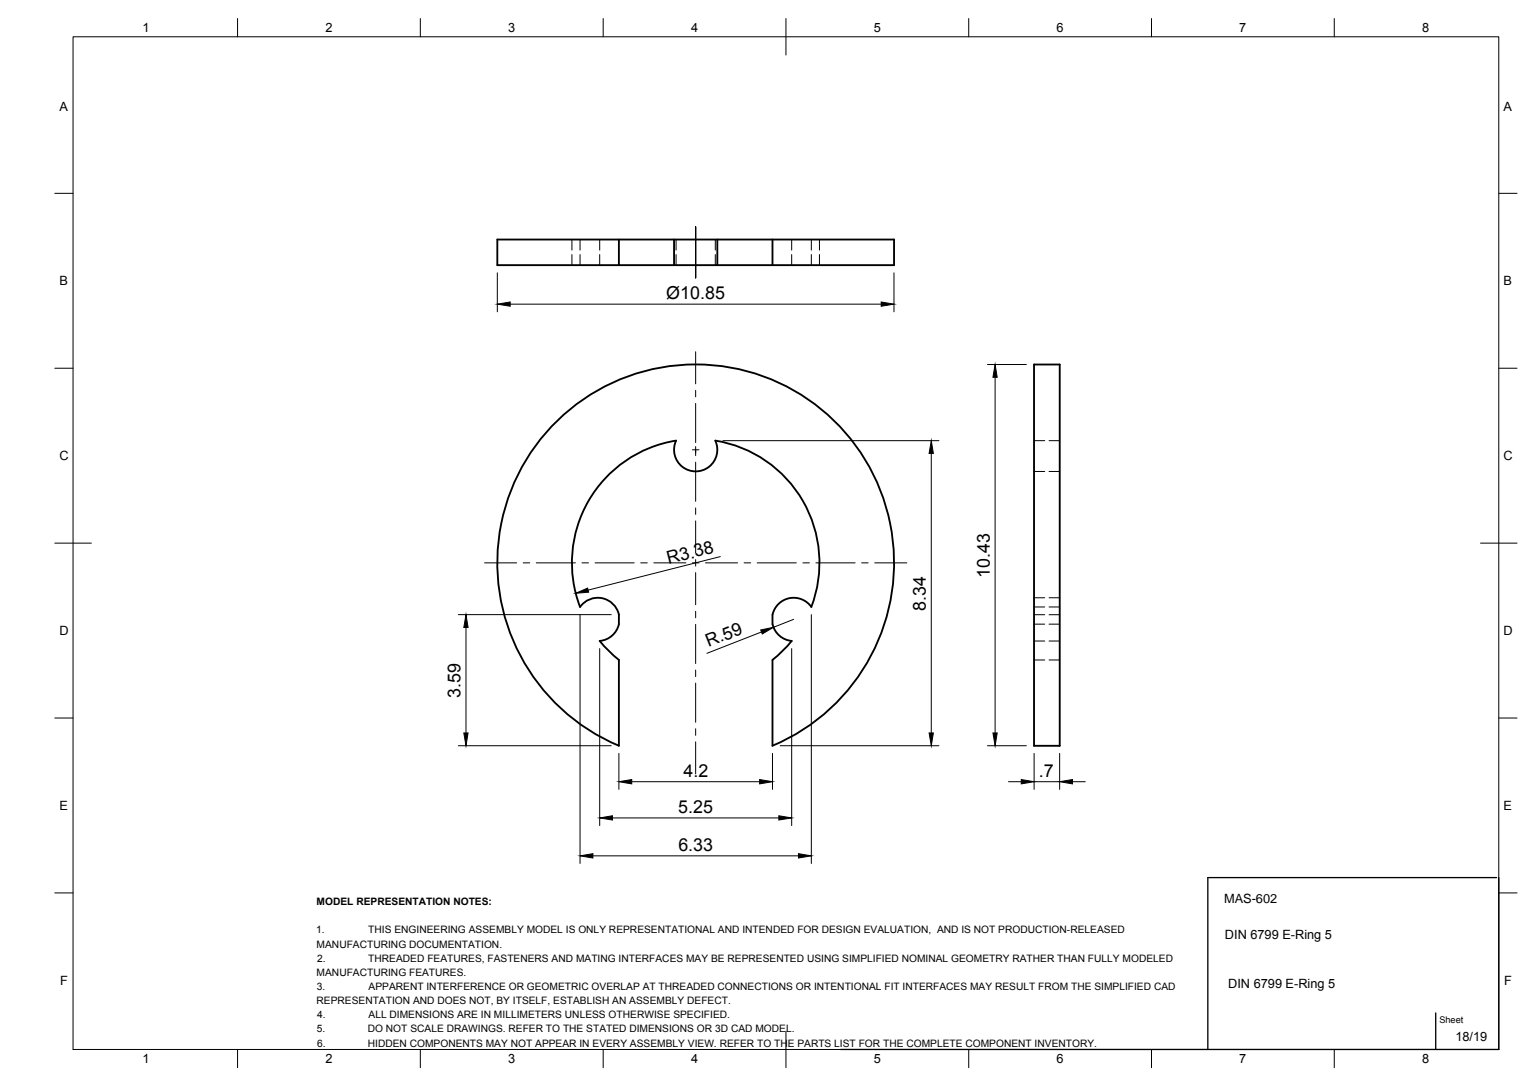
ISO-10303-21;
HEADER;
/* Generated by software containing ST-Developer
 * from STEP Tools, Inc. (www.steptools.com) 
 */

FILE_DESCRIPTION(
/* description */ (''),
/* implementation_level */ '2;1');

FILE_NAME(
/* name */ 'DIN 6799 E-Ring 5.step',
/* time_stamp */ '2026-10-15T14:42:47-07:00',
/* author */ (''),
/* organization */ (''),
/* preprocessor_version */ 'ST-DEVELOPER v20.2',
/* originating_system */ 'Autodesk Translation Framework v15.15.0.0',
/* authorisation */ '');

FILE_SCHEMA (('AUTOMOTIVE_DESIGN { 1 0 10303 214 3 1 1 }'));
ENDSEC;

DATA;
#10=MECHANICAL_DESIGN_GEOMETRIC_PRESENTATION_REPRESENTATION('',(#250),#85789);
#214=SHAPE_REPRESENTATION_RELATIONSHIP('SRR','None',#85879,#232);
#232=ADVANCED_BREP_SHAPE_REPRESENTATION('',(#268),#85787);
#250=STYLED_ITEM('',(#85978),#268);
#268=MANIFOLD_SOLID_BREP('Body1',#9897);
#1187=PLANE('',#10856);
#1188=PLANE('',#10857);
#1189=PLANE('',#10858);
#1190=PLANE('',#10859);
#1191=PLANE('',#10875);
#1192=PLANE('',#10891);
#1691=LINE('',#85550,#2227);
#1692=LINE('',#85552,#2228);
#1693=LINE('',#85554,#2229);
#1694=LINE('',#85555,#2230);
#1695=LINE('',#85559,#2231);
#1696=LINE('',#85561,#2232);
#1697=LINE('',#85563,#2233);
#1698=LINE('',#85564,#2234);
#1699=LINE('',#85568,#2235);
#1700=LINE('',#85570,#2236);
#1701=LINE('',#85572,#2237);
#1702=LINE('',#85573,#2238);
#1703=LINE('',#85577,#2239);
#1704=LINE('',#85579,#2240);
#1705=LINE('',#85581,#2241);
#1706=LINE('',#85582,#2242);
#1707=LINE('',#85587,#2243);
#1708=LINE('',#85593,#2244);
#1709=LINE('',#85599,#2245);
#1710=LINE('',#85605,#2246);
#1711=LINE('',#85623,#2247);
#1712=LINE('',#85627,#2248);
#2227=VECTOR('',#12969,1.);
#2228=VECTOR('',#12970,1.);
#2229=VECTOR('',#12971,1.);
#2230=VECTOR('',#12972,1.);
#2231=VECTOR('',#12975,1.);
#2232=VECTOR('',#12976,1.);
#2233=VECTOR('',#12977,1.);
#2234=VECTOR('',#12978,1.);
#2235=VECTOR('',#12981,1.);
#2236=VECTOR('',#12982,1.);
#2237=VECTOR('',#12983,1.);
#2238=VECTOR('',#12984,1.);
#2239=VECTOR('',#12987,1.);
#2240=VECTOR('',#12988,1.);
#2241=VECTOR('',#12989,1.);
#2242=VECTOR('',#12990,1.);
#2243=VECTOR('',#12995,1.);
#2244=VECTOR('',#13002,1.);
#2245=VECTOR('',#13009,1.);
#2246=VECTOR('',#13016,1.);
#2247=VECTOR('',#13045,1.);
#2248=VECTOR('',#13050,1.);
#2382=CYLINDRICAL_SURFACE('',#10860,0.059240625);
#2383=CYLINDRICAL_SURFACE('',#10863,0.059240625);
#2384=CYLINDRICAL_SURFACE('',#10866,0.059240625);
#2385=CYLINDRICAL_SURFACE('',#10869,0.059240625);
#2386=CYLINDRICAL_SURFACE('',#10872,0.33848125);
#2387=CYLINDRICAL_SURFACE('',#10881,0.33848125);
#2388=CYLINDRICAL_SURFACE('',#10883,0.33848125);
#2389=CYLINDRICAL_SURFACE('',#10885,0.059240625);
#2390=CYLINDRICAL_SURFACE('',#10887,0.33848125);
#2391=CYLINDRICAL_SURFACE('',#10889,0.5425);
#2871=FACE_OUTER_BOUND('',#3461,.T.);
#2872=FACE_OUTER_BOUND('',#3462,.T.);
#2873=FACE_OUTER_BOUND('',#3463,.T.);
#2874=FACE_OUTER_BOUND('',#3464,.T.);
#2875=FACE_OUTER_BOUND('',#3465,.T.);
#2876=FACE_OUTER_BOUND('',#3466,.T.);
#2877=FACE_OUTER_BOUND('',#3467,.T.);
#2878=FACE_OUTER_BOUND('',#3468,.T.);
#2879=FACE_OUTER_BOUND('',#3469,.T.);
#2880=FACE_OUTER_BOUND('',#3470,.T.);
#2881=FACE_OUTER_BOUND('',#3471,.T.);
#2882=FACE_OUTER_BOUND('',#3472,.T.);
#2883=FACE_OUTER_BOUND('',#3473,.T.);
#2884=FACE_OUTER_BOUND('',#3474,.T.);
#2885=FACE_OUTER_BOUND('',#3475,.T.);
#2886=FACE_OUTER_BOUND('',#3476,.T.);
#3461=EDGE_LOOP('',(#9207,#9208,#9209,#9210));
#3462=EDGE_LOOP('',(#9211,#9212,#9213,#9214));
#3463=EDGE_LOOP('',(#9215,#9216,#9217,#9218));
#3464=EDGE_LOOP('',(#9219,#9220,#9221,#9222));
#3465=EDGE_LOOP('',(#9223,#9224,#9225,#9226));
#3466=EDGE_LOOP('',(#9227,#9228,#9229,#9230));
#3467=EDGE_LOOP('',(#9231,#9232,#9233,#9234));
#3468=EDGE_LOOP('',(#9235,#9236,#9237,#9238));
#3469=EDGE_LOOP('',(#9239,#9240,#9241,#9242));
#3470=EDGE_LOOP('',(#9243,#9244,#9245,#9246,#9247,#9248,#9249,#9250,#9251,
#9252,#9253,#9254,#9255,#9256));
#3471=EDGE_LOOP('',(#9257,#9258,#9259,#9260));
#3472=EDGE_LOOP('',(#9261,#9262,#9263,#9264));
#3473=EDGE_LOOP('',(#9265,#9266,#9267,#9268));
#3474=EDGE_LOOP('',(#9269,#9270,#9271,#9272));
#3475=EDGE_LOOP('',(#9273,#9274,#9275,#9276));
#3476=EDGE_LOOP('',(#9277,#9278,#9279,#9280,#9281,#9282,#9283,#9284,#9285,
#9286,#9287,#9288,#9289,#9290));
#3855=CIRCLE('',#10861,0.059240625);
#3856=CIRCLE('',#10862,0.059240625);
#3857=CIRCLE('',#10864,0.059240625);
#3858=CIRCLE('',#10865,0.059240625);
#3859=CIRCLE('',#10867,0.059240625);
#3860=CIRCLE('',#10868,0.059240625);
#3861=CIRCLE('',#10870,0.059240625);
#3862=CIRCLE('',#10871,0.059240625);
#3863=CIRCLE('',#10873,0.33848125);
#3864=CIRCLE('',#10874,0.33848125);
#3865=CIRCLE('',#10876,0.33848125);
#3866=CIRCLE('',#10877,0.059240625);
#3867=CIRCLE('',#10878,0.33848125);
#3868=CIRCLE('',#10879,0.5425);
#3869=CIRCLE('',#10880,0.33848125);
#3870=CIRCLE('',#10882,0.33848125);
#3871=CIRCLE('',#10884,0.33848125);
#3872=CIRCLE('',#10886,0.059240625);
#3873=CIRCLE('',#10888,0.33848125);
#3874=CIRCLE('',#10890,0.5425);
#4879=VERTEX_POINT('',#85548);
#4880=VERTEX_POINT('',#85549);
#4881=VERTEX_POINT('',#85551);
#4882=VERTEX_POINT('',#85553);
#4883=VERTEX_POINT('',#85557);
#4884=VERTEX_POINT('',#85558);
#4885=VERTEX_POINT('',#85560);
#4886=VERTEX_POINT('',#85562);
#4887=VERTEX_POINT('',#85566);
#4888=VERTEX_POINT('',#85567);
#4889=VERTEX_POINT('',#85569);
#4890=VERTEX_POINT('',#85571);
#4891=VERTEX_POINT('',#85575);
#4892=VERTEX_POINT('',#85576);
#4893=VERTEX_POINT('',#85578);
#4894=VERTEX_POINT('',#85580);
#4895=VERTEX_POINT('',#85584);
#4896=VERTEX_POINT('',#85586);
#4897=VERTEX_POINT('',#85590);
#4898=VERTEX_POINT('',#85592);
#4899=VERTEX_POINT('',#85596);
#4900=VERTEX_POINT('',#85598);
#4901=VERTEX_POINT('',#85602);
#4902=VERTEX_POINT('',#85604);
#4903=VERTEX_POINT('',#85611);
#4904=VERTEX_POINT('',#85613);
#4905=VERTEX_POINT('',#85621);
#4906=VERTEX_POINT('',#85625);
#6331=EDGE_CURVE('',#4879,#4880,#1691,.T.);
#6332=EDGE_CURVE('',#4881,#4879,#1692,.T.);
#6333=EDGE_CURVE('',#4882,#4881,#1693,.T.);
#6334=EDGE_CURVE('',#4880,#4882,#1694,.T.);
#6335=EDGE_CURVE('',#4883,#4884,#1695,.T.);
#6336=EDGE_CURVE('',#4885,#4883,#1696,.T.);
#6337=EDGE_CURVE('',#4886,#4885,#1697,.T.);
#6338=EDGE_CURVE('',#4884,#4886,#1698,.T.);
#6339=EDGE_CURVE('',#4887,#4888,#1699,.T.);
#6340=EDGE_CURVE('',#4889,#4887,#1700,.T.);
#6341=EDGE_CURVE('',#4890,#4889,#1701,.T.);
#6342=EDGE_CURVE('',#4888,#4890,#1702,.T.);
#6343=EDGE_CURVE('',#4891,#4892,#1703,.T.);
#6344=EDGE_CURVE('',#4893,#4891,#1704,.T.);
#6345=EDGE_CURVE('',#4894,#4893,#1705,.T.);
#6346=EDGE_CURVE('',#4892,#4894,#1706,.T.);
#6347=EDGE_CURVE('',#4895,#4885,#3855,.T.);
#6348=EDGE_CURVE('',#4896,#4895,#1707,.T.);
#6349=EDGE_CURVE('',#4896,#4886,#3856,.T.);
#6350=EDGE_CURVE('',#4884,#4897,#3857,.T.);
#6351=EDGE_CURVE('',#4897,#4898,#1708,.T.);
#6352=EDGE_CURVE('',#4883,#4898,#3858,.T.);
#6353=EDGE_CURVE('',#4899,#4893,#3859,.T.);
#6354=EDGE_CURVE('',#4900,#4899,#1709,.T.);
#6355=EDGE_CURVE('',#4900,#4894,#3860,.T.);
#6356=EDGE_CURVE('',#4892,#4901,#3861,.T.);
#6357=EDGE_CURVE('',#4901,#4902,#1710,.T.);
#6358=EDGE_CURVE('',#4891,#4902,#3862,.T.);
#6359=EDGE_CURVE('',#4888,#4900,#3863,.T.);
#6360=EDGE_CURVE('',#4887,#4899,#3864,.T.);
#6361=EDGE_CURVE('',#4903,#4896,#3865,.T.);
#6362=EDGE_CURVE('',#4904,#4903,#3866,.T.);
#6363=EDGE_CURVE('',#4901,#4904,#3867,.T.);
#6364=EDGE_CURVE('',#4881,#4890,#3868,.T.);
#6365=EDGE_CURVE('',#4897,#4879,#3869,.T.);
#6366=EDGE_CURVE('',#4898,#4880,#3870,.T.);
#6367=EDGE_CURVE('',#4905,#4895,#3871,.T.);
#6368=EDGE_CURVE('',#4903,#4905,#1711,.T.);
#6369=EDGE_CURVE('',#4906,#4905,#3872,.T.);
#6370=EDGE_CURVE('',#4904,#4906,#1712,.T.);
#6371=EDGE_CURVE('',#4902,#4906,#3873,.T.);
#6372=EDGE_CURVE('',#4882,#4889,#3874,.T.);
#9207=ORIENTED_EDGE('',*,*,#6331,.F.);
#9208=ORIENTED_EDGE('',*,*,#6332,.F.);
#9209=ORIENTED_EDGE('',*,*,#6333,.F.);
#9210=ORIENTED_EDGE('',*,*,#6334,.F.);
#9211=ORIENTED_EDGE('',*,*,#6335,.F.);
#9212=ORIENTED_EDGE('',*,*,#6336,.F.);
#9213=ORIENTED_EDGE('',*,*,#6337,.F.);
#9214=ORIENTED_EDGE('',*,*,#6338,.F.);
#9215=ORIENTED_EDGE('',*,*,#6339,.F.);
#9216=ORIENTED_EDGE('',*,*,#6340,.F.);
#9217=ORIENTED_EDGE('',*,*,#6341,.F.);
#9218=ORIENTED_EDGE('',*,*,#6342,.F.);
#9219=ORIENTED_EDGE('',*,*,#6343,.F.);
#9220=ORIENTED_EDGE('',*,*,#6344,.F.);
#9221=ORIENTED_EDGE('',*,*,#6345,.F.);
#9222=ORIENTED_EDGE('',*,*,#6346,.F.);
#9223=ORIENTED_EDGE('',*,*,#6337,.T.);
#9224=ORIENTED_EDGE('',*,*,#6347,.F.);
#9225=ORIENTED_EDGE('',*,*,#6348,.F.);
#9226=ORIENTED_EDGE('',*,*,#6349,.T.);
#9227=ORIENTED_EDGE('',*,*,#6335,.T.);
#9228=ORIENTED_EDGE('',*,*,#6350,.T.);
#9229=ORIENTED_EDGE('',*,*,#6351,.T.);
#9230=ORIENTED_EDGE('',*,*,#6352,.F.);
#9231=ORIENTED_EDGE('',*,*,#6345,.T.);
#9232=ORIENTED_EDGE('',*,*,#6353,.F.);
#9233=ORIENTED_EDGE('',*,*,#6354,.F.);
#9234=ORIENTED_EDGE('',*,*,#6355,.T.);
#9235=ORIENTED_EDGE('',*,*,#6343,.T.);
#9236=ORIENTED_EDGE('',*,*,#6356,.T.);
#9237=ORIENTED_EDGE('',*,*,#6357,.T.);
#9238=ORIENTED_EDGE('',*,*,#6358,.F.);
#9239=ORIENTED_EDGE('',*,*,#6339,.T.);
#9240=ORIENTED_EDGE('',*,*,#6359,.T.);
#9241=ORIENTED_EDGE('',*,*,#6354,.T.);
#9242=ORIENTED_EDGE('',*,*,#6360,.F.);
#9243=ORIENTED_EDGE('',*,*,#6338,.T.);
#9244=ORIENTED_EDGE('',*,*,#6349,.F.);
#9245=ORIENTED_EDGE('',*,*,#6361,.F.);
#9246=ORIENTED_EDGE('',*,*,#6362,.F.);
#9247=ORIENTED_EDGE('',*,*,#6363,.F.);
#9248=ORIENTED_EDGE('',*,*,#6356,.F.);
#9249=ORIENTED_EDGE('',*,*,#6346,.T.);
#9250=ORIENTED_EDGE('',*,*,#6355,.F.);
#9251=ORIENTED_EDGE('',*,*,#6359,.F.);
#9252=ORIENTED_EDGE('',*,*,#6342,.T.);
#9253=ORIENTED_EDGE('',*,*,#6364,.F.);
#9254=ORIENTED_EDGE('',*,*,#6332,.T.);
#9255=ORIENTED_EDGE('',*,*,#6365,.F.);
#9256=ORIENTED_EDGE('',*,*,#6350,.F.);
#9257=ORIENTED_EDGE('',*,*,#6331,.T.);
#9258=ORIENTED_EDGE('',*,*,#6366,.F.);
#9259=ORIENTED_EDGE('',*,*,#6351,.F.);
#9260=ORIENTED_EDGE('',*,*,#6365,.T.);
#9261=ORIENTED_EDGE('',*,*,#6361,.T.);
#9262=ORIENTED_EDGE('',*,*,#6348,.T.);
#9263=ORIENTED_EDGE('',*,*,#6367,.F.);
#9264=ORIENTED_EDGE('',*,*,#6368,.F.);
#9265=ORIENTED_EDGE('',*,*,#6362,.T.);
#9266=ORIENTED_EDGE('',*,*,#6368,.T.);
#9267=ORIENTED_EDGE('',*,*,#6369,.F.);
#9268=ORIENTED_EDGE('',*,*,#6370,.F.);
#9269=ORIENTED_EDGE('',*,*,#6363,.T.);
#9270=ORIENTED_EDGE('',*,*,#6370,.T.);
#9271=ORIENTED_EDGE('',*,*,#6371,.F.);
#9272=ORIENTED_EDGE('',*,*,#6357,.F.);
#9273=ORIENTED_EDGE('',*,*,#6333,.T.);
#9274=ORIENTED_EDGE('',*,*,#6364,.T.);
#9275=ORIENTED_EDGE('',*,*,#6341,.T.);
#9276=ORIENTED_EDGE('',*,*,#6372,.F.);
#9277=ORIENTED_EDGE('',*,*,#6336,.T.);
#9278=ORIENTED_EDGE('',*,*,#6352,.T.);
#9279=ORIENTED_EDGE('',*,*,#6366,.T.);
#9280=ORIENTED_EDGE('',*,*,#6334,.T.);
#9281=ORIENTED_EDGE('',*,*,#6372,.T.);
#9282=ORIENTED_EDGE('',*,*,#6340,.T.);
#9283=ORIENTED_EDGE('',*,*,#6360,.T.);
#9284=ORIENTED_EDGE('',*,*,#6353,.T.);
#9285=ORIENTED_EDGE('',*,*,#6344,.T.);
#9286=ORIENTED_EDGE('',*,*,#6358,.T.);
#9287=ORIENTED_EDGE('',*,*,#6371,.T.);
#9288=ORIENTED_EDGE('',*,*,#6369,.T.);
#9289=ORIENTED_EDGE('',*,*,#6367,.T.);
#9290=ORIENTED_EDGE('',*,*,#6347,.T.);
#9849=ADVANCED_FACE('',(#2871),#1187,.F.);
#9850=ADVANCED_FACE('',(#2872),#1188,.F.);
#9851=ADVANCED_FACE('',(#2873),#1189,.F.);
#9852=ADVANCED_FACE('',(#2874),#1190,.F.);
#9853=ADVANCED_FACE('',(#2875),#2382,.T.);
#9854=ADVANCED_FACE('',(#2876),#2383,.T.);
#9855=ADVANCED_FACE('',(#2877),#2384,.T.);
#9856=ADVANCED_FACE('',(#2878),#2385,.T.);
#9857=ADVANCED_FACE('',(#2879),#2386,.F.);
#9858=ADVANCED_FACE('',(#2880),#1191,.F.);
#9859=ADVANCED_FACE('',(#2881),#2387,.F.);
#9860=ADVANCED_FACE('',(#2882),#2388,.F.);
#9861=ADVANCED_FACE('',(#2883),#2389,.T.);
#9862=ADVANCED_FACE('',(#2884),#2390,.F.);
#9863=ADVANCED_FACE('',(#2885),#2391,.T.);
#9864=ADVANCED_FACE('',(#2886),#1192,.T.);
#9897=CLOSED_SHELL('',(#9849,#9850,#9851,#9852,#9853,#9854,#9855,#9856,
#9857,#9858,#9859,#9860,#9861,#9862,#9863,#9864));
#10855=AXIS2_PLACEMENT_3D('',#85546,#12965,#12966);
#10856=AXIS2_PLACEMENT_3D('',#85547,#12967,#12968);
#10857=AXIS2_PLACEMENT_3D('',#85556,#12973,#12974);
#10858=AXIS2_PLACEMENT_3D('',#85565,#12979,#12980);
#10859=AXIS2_PLACEMENT_3D('',#85574,#12985,#12986);
#10860=AXIS2_PLACEMENT_3D('',#85583,#12991,#12992);
#10861=AXIS2_PLACEMENT_3D('',#85585,#12993,#12994);
#10862=AXIS2_PLACEMENT_3D('',#85588,#12996,#12997);
#10863=AXIS2_PLACEMENT_3D('',#85589,#12998,#12999);
#10864=AXIS2_PLACEMENT_3D('',#85591,#13000,#13001);
#10865=AXIS2_PLACEMENT_3D('',#85594,#13003,#13004);
#10866=AXIS2_PLACEMENT_3D('',#85595,#13005,#13006);
#10867=AXIS2_PLACEMENT_3D('',#85597,#13007,#13008);
#10868=AXIS2_PLACEMENT_3D('',#85600,#13010,#13011);
#10869=AXIS2_PLACEMENT_3D('',#85601,#13012,#13013);
#10870=AXIS2_PLACEMENT_3D('',#85603,#13014,#13015);
#10871=AXIS2_PLACEMENT_3D('',#85606,#13017,#13018);
#10872=AXIS2_PLACEMENT_3D('',#85607,#13019,#13020);
#10873=AXIS2_PLACEMENT_3D('',#85608,#13021,#13022);
#10874=AXIS2_PLACEMENT_3D('',#85609,#13023,#13024);
#10875=AXIS2_PLACEMENT_3D('',#85610,#13025,#13026);
#10876=AXIS2_PLACEMENT_3D('',#85612,#13027,#13028);
#10877=AXIS2_PLACEMENT_3D('',#85614,#13029,#13030);
#10878=AXIS2_PLACEMENT_3D('',#85615,#13031,#13032);
#10879=AXIS2_PLACEMENT_3D('',#85616,#13033,#13034);
#10880=AXIS2_PLACEMENT_3D('',#85617,#13035,#13036);
#10881=AXIS2_PLACEMENT_3D('',#85618,#13037,#13038);
#10882=AXIS2_PLACEMENT_3D('',#85619,#13039,#13040);
#10883=AXIS2_PLACEMENT_3D('',#85620,#13041,#13042);
#10884=AXIS2_PLACEMENT_3D('',#85622,#13043,#13044);
#10885=AXIS2_PLACEMENT_3D('',#85624,#13046,#13047);
#10886=AXIS2_PLACEMENT_3D('',#85626,#13048,#13049);
#10887=AXIS2_PLACEMENT_3D('',#85628,#13051,#13052);
#10888=AXIS2_PLACEMENT_3D('',#85629,#13053,#13054);
#10889=AXIS2_PLACEMENT_3D('',#85630,#13055,#13056);
#10890=AXIS2_PLACEMENT_3D('',#85631,#13057,#13058);
#10891=AXIS2_PLACEMENT_3D('',#85632,#13059,#13060);
#12965=DIRECTION('axis',(0.,0.,1.));
#12966=DIRECTION('refdir',(1.,0.,0.));
#12967=DIRECTION('center_axis',(0.,1.,0.));
#12968=DIRECTION('ref_axis',(0.,0.,1.));
#12969=DIRECTION('',(1.,0.,0.));
#12970=DIRECTION('',(0.,0.,1.));
#12971=DIRECTION('',(-1.,0.,0.));
#12972=DIRECTION('',(0.,0.,-1.));
#12973=DIRECTION('center_axis',(0.,1.,0.));
#12974=DIRECTION('ref_axis',(0.,0.,1.));
#12975=DIRECTION('',(-1.,0.,0.));
#12976=DIRECTION('',(0.,0.,-1.));
#12977=DIRECTION('',(1.,0.,0.));
#12978=DIRECTION('',(0.,0.,1.));
#12979=DIRECTION('center_axis',(0.,-1.,0.));
#12980=DIRECTION('ref_axis',(0.,0.,-1.));
#12981=DIRECTION('',(-1.,0.,0.));
#12982=DIRECTION('',(0.,0.,1.));
#12983=DIRECTION('',(1.,0.,0.));
#12984=DIRECTION('',(0.,0.,-1.));
#12985=DIRECTION('center_axis',(0.,-1.,0.));
#12986=DIRECTION('ref_axis',(0.,0.,-1.));
#12987=DIRECTION('',(-1.,0.,0.));
#12988=DIRECTION('',(0.,0.,1.));
#12989=DIRECTION('',(1.,0.,0.));
#12990=DIRECTION('',(0.,0.,-1.));
#12991=DIRECTION('center_axis',(1.,0.,0.));
#12992=DIRECTION('ref_axis',(0.,-0.194892865217565,0.980824536340363));
#12993=DIRECTION('center_axis',(1.,0.,0.));
#12994=DIRECTION('ref_axis',(0.,0.,-1.));
#12995=DIRECTION('',(1.,0.,0.));
#12996=DIRECTION('center_axis',(1.,0.,0.));
#12997=DIRECTION('ref_axis',(0.,0.,-1.));
#12998=DIRECTION('center_axis',(1.,0.,0.));
#12999=DIRECTION('ref_axis',(0.,0.,-1.));
#13000=DIRECTION('center_axis',(1.,0.,0.));
#13001=DIRECTION('ref_axis',(0.,0.,-1.));
#13002=DIRECTION('',(1.,0.,0.));
#13003=DIRECTION('center_axis',(1.,0.,0.));
#13004=DIRECTION('ref_axis',(0.,0.,-1.));
#13005=DIRECTION('center_axis',(1.,0.,0.));
#13006=DIRECTION('ref_axis',(0.,0.,-1.));
#13007=DIRECTION('center_axis',(1.,0.,0.));
#13008=DIRECTION('ref_axis',(0.,0.,-1.));
#13009=DIRECTION('',(1.,0.,0.));
#13010=DIRECTION('center_axis',(1.,0.,0.));
#13011=DIRECTION('ref_axis',(0.,0.,-1.));
#13012=DIRECTION('center_axis',(1.,0.,0.));
#13013=DIRECTION('ref_axis',(0.,0.194892865217571,0.980824536340362));
#13014=DIRECTION('center_axis',(1.,0.,0.));
#13015=DIRECTION('ref_axis',(0.,0.,-1.));
#13016=DIRECTION('',(1.,0.,0.));
#13017=DIRECTION('center_axis',(1.,0.,0.));
#13018=DIRECTION('ref_axis',(0.,0.,-1.));
#13019=DIRECTION('center_axis',(1.,0.,0.));
#13020=DIRECTION('ref_axis',(0.,0.,-1.));
#13021=DIRECTION('center_axis',(-1.,0.,0.));
#13022=DIRECTION('ref_axis',(0.,0.,-1.));
#13023=DIRECTION('center_axis',(-1.,0.,0.));
#13024=DIRECTION('ref_axis',(0.,0.,-1.));
#13025=DIRECTION('center_axis',(1.,0.,0.));
#13026=DIRECTION('ref_axis',(0.,0.,-1.));
#13027=DIRECTION('center_axis',(-1.,0.,0.));
#13028=DIRECTION('ref_axis',(0.,0.,-1.));
#13029=DIRECTION('center_axis',(1.,0.,0.));
#13030=DIRECTION('ref_axis',(0.,0.,-1.));
#13031=DIRECTION('center_axis',(-1.,0.,0.));
#13032=DIRECTION('ref_axis',(0.,0.,-1.));
#13033=DIRECTION('center_axis',(1.,0.,0.));
#13034=DIRECTION('ref_axis',(0.,0.,-1.));
#13035=DIRECTION('center_axis',(-1.,0.,0.));
#13036=DIRECTION('ref_axis',(0.,0.,-1.));
#13037=DIRECTION('center_axis',(1.,0.,0.));
#13038=DIRECTION('ref_axis',(0.,0.,-1.));
#13039=DIRECTION('center_axis',(-1.,0.,0.));
#13040=DIRECTION('ref_axis',(0.,0.,-1.));
#13041=DIRECTION('center_axis',(1.,0.,0.));
#13042=DIRECTION('ref_axis',(0.,0.,-1.));
#13043=DIRECTION('center_axis',(-1.,0.,0.));
#13044=DIRECTION('ref_axis',(0.,0.,-1.));
#13045=DIRECTION('',(1.,0.,0.));
#13046=DIRECTION('center_axis',(1.,0.,0.));
#13047=DIRECTION('ref_axis',(0.,0.,-1.));
#13048=DIRECTION('center_axis',(1.,0.,0.));
#13049=DIRECTION('ref_axis',(0.,0.,-1.));
#13050=DIRECTION('',(1.,0.,0.));
#13051=DIRECTION('center_axis',(1.,0.,0.));
#13052=DIRECTION('ref_axis',(0.,0.,-1.));
#13053=DIRECTION('center_axis',(-1.,0.,0.));
#13054=DIRECTION('ref_axis',(0.,0.,-1.));
#13055=DIRECTION('center_axis',(1.,0.,0.));
#13056=DIRECTION('ref_axis',(0.,1.22464679914735E-16,1.));
#13057=DIRECTION('center_axis',(1.,0.,0.));
#13058=DIRECTION('ref_axis',(0.,0.,-1.));
#13059=DIRECTION('center_axis',(1.,0.,0.));
#13060=DIRECTION('ref_axis',(0.,0.,-1.));
#85546=CARTESIAN_POINT('',(0.,0.,0.));
#85547=CARTESIAN_POINT('Origin',(0.,0.21,-1.085));
#85548=CARTESIAN_POINT('',(0.,0.21,-0.265461026520961));
#85549=CARTESIAN_POINT('',(0.07,0.21,-0.265461026520961));
#85550=CARTESIAN_POINT('',(0.,0.21,-0.265461026520961));
#85551=CARTESIAN_POINT('',(0.,0.21,-0.500206207478476));
#85552=CARTESIAN_POINT('',(0.,0.21,-0.5425));
#85553=CARTESIAN_POINT('',(0.07,0.21,-0.500206207478476));
#85554=CARTESIAN_POINT('',(0.,0.21,-0.500206207478476));
#85555=CARTESIAN_POINT('',(0.07,0.21,-0.5425));
#85556=CARTESIAN_POINT('Origin',(0.,0.21,-1.085));
#85557=CARTESIAN_POINT('',(0.07,0.21,-0.167559714847562));
#85558=CARTESIAN_POINT('',(0.,0.21,-0.167559714847562));
#85559=CARTESIAN_POINT('',(0.,0.21,-0.167559714847562));
#85560=CARTESIAN_POINT('',(0.07,0.21,-0.141680910152439));
#85561=CARTESIAN_POINT('',(0.07,0.21,-0.5425));
#85562=CARTESIAN_POINT('',(0.,0.21,-0.141680910152439));
#85563=CARTESIAN_POINT('',(0.,0.21,-0.141680910152439));
#85564=CARTESIAN_POINT('',(0.,0.21,-0.5425));
#85565=CARTESIAN_POINT('Origin',(0.,-0.21,-0.075));
#85566=CARTESIAN_POINT('',(0.07,-0.21,-0.265461026520961));
#85567=CARTESIAN_POINT('',(0.,-0.21,-0.265461026520961));
#85568=CARTESIAN_POINT('',(0.,-0.21,-0.265461026520961));
#85569=CARTESIAN_POINT('',(0.07,-0.21,-0.500206207478476));
#85570=CARTESIAN_POINT('',(0.07,-0.21,-0.0375));
#85571=CARTESIAN_POINT('',(0.,-0.21,-0.500206207478476));
#85572=CARTESIAN_POINT('',(0.,-0.21,-0.500206207478476));
#85573=CARTESIAN_POINT('',(0.,-0.21,-0.0375));
#85574=CARTESIAN_POINT('Origin',(0.,-0.21,-0.075));
#85575=CARTESIAN_POINT('',(0.07,-0.21,-0.141680910152439));
#85576=CARTESIAN_POINT('',(0.,-0.21,-0.141680910152439));
#85577=CARTESIAN_POINT('',(0.,-0.21,-0.141680910152439));
#85578=CARTESIAN_POINT('',(0.07,-0.21,-0.167559714847561));
#85579=CARTESIAN_POINT('',(0.07,-0.21,-0.0375));
#85580=CARTESIAN_POINT('',(0.,-0.21,-0.167559714847561));
#85581=CARTESIAN_POINT('',(0.,-0.21,-0.167559714847561));
#85582=CARTESIAN_POINT('',(0.,-0.21,-0.0375));
#85583=CARTESIAN_POINT('Origin',(0.,0.267810237132177,-0.1546203125));
#85584=CARTESIAN_POINT('',(0.07,0.31628195418898,-0.120562357541491));
#85585=CARTESIAN_POINT('Origin',(0.07,0.267810237132177,-0.1546203125));
#85586=CARTESIAN_POINT('',(0.,0.31628195418898,-0.120562357541491));
#85587=CARTESIAN_POINT('',(0.,0.31628195418898,-0.120562357541491));
#85588=CARTESIAN_POINT('Origin',(0.,0.267810237132177,-0.1546203125));
#85589=CARTESIAN_POINT('Origin',(0.,0.267810237132177,-0.1546203125));
#85590=CARTESIAN_POINT('',(0.,0.262551041465563,-0.213627028315498));
#85591=CARTESIAN_POINT('Origin',(0.,0.267810237132177,-0.1546203125));
#85592=CARTESIAN_POINT('',(0.07,0.262551041465563,-0.213627028315498));
#85593=CARTESIAN_POINT('',(0.,0.262551041465563,-0.213627028315498));
#85594=CARTESIAN_POINT('Origin',(0.07,0.267810237132177,-0.1546203125));
#85595=CARTESIAN_POINT('Origin',(0.,-0.267810237132177,-0.1546203125));
#85596=CARTESIAN_POINT('',(0.07,-0.262551041465564,-0.213627028315498));
#85597=CARTESIAN_POINT('Origin',(0.07,-0.267810237132177,-0.1546203125));
#85598=CARTESIAN_POINT('',(0.,-0.262551041465564,-0.213627028315498));
#85599=CARTESIAN_POINT('',(0.,-0.262551041465564,-0.213627028315498));
#85600=CARTESIAN_POINT('Origin',(0.,-0.267810237132177,-0.1546203125));
#85601=CARTESIAN_POINT('Origin',(0.,-0.267810237132177,-0.1546203125));
#85602=CARTESIAN_POINT('',(0.,-0.31628195418898,-0.120562357541491));
#85603=CARTESIAN_POINT('Origin',(0.,-0.267810237132177,-0.1546203125));
#85604=CARTESIAN_POINT('',(0.07,-0.31628195418898,-0.120562357541491));
#85605=CARTESIAN_POINT('',(0.,-0.31628195418898,-0.120562357541491));
#85606=CARTESIAN_POINT('Origin',(0.07,-0.267810237132177,-0.1546203125));
#85607=CARTESIAN_POINT('Origin',(0.,0.,0.));
#85608=CARTESIAN_POINT('Origin',(0.,0.,0.));
#85609=CARTESIAN_POINT('Origin',(0.07,0.,0.));
#85610=CARTESIAN_POINT('Origin',(0.,0.,0.));
#85611=CARTESIAN_POINT('',(0.,0.0537309127234168,0.334189385856988));
#85612=CARTESIAN_POINT('Origin',(0.,0.,0.));
#85613=CARTESIAN_POINT('',(0.,-0.0537309127234167,0.334189385856988));
#85614=CARTESIAN_POINT('Origin',(0.,1.89355270786289E-17,0.309240625));
#85615=CARTESIAN_POINT('Origin',(0.,0.,0.));
#85616=CARTESIAN_POINT('Origin',(0.,0.,0.));
#85617=CARTESIAN_POINT('Origin',(0.,0.,0.));
#85618=CARTESIAN_POINT('Origin',(0.,0.,0.));
#85619=CARTESIAN_POINT('Origin',(0.07,0.,0.));
#85620=CARTESIAN_POINT('Origin',(0.,0.,0.));
#85621=CARTESIAN_POINT('',(0.07,0.0537309127234168,0.334189385856988));
#85622=CARTESIAN_POINT('Origin',(0.07,0.,0.));
#85623=CARTESIAN_POINT('',(0.,0.0537309127234168,0.334189385856988));
#85624=CARTESIAN_POINT('Origin',(0.,1.89355270786289E-17,0.309240625));
#85625=CARTESIAN_POINT('',(0.07,-0.0537309127234167,0.334189385856988));
#85626=CARTESIAN_POINT('Origin',(0.07,1.89355270786289E-17,0.309240625));
#85627=CARTESIAN_POINT('',(0.,-0.0537309127234167,0.334189385856988));
#85628=CARTESIAN_POINT('Origin',(0.,0.,0.));
#85629=CARTESIAN_POINT('Origin',(0.07,0.,0.));
#85630=CARTESIAN_POINT('Origin',(0.,0.,0.));
#85631=CARTESIAN_POINT('Origin',(0.07,0.,0.));
#85632=CARTESIAN_POINT('Origin',(0.07,0.,0.));
#85767=UNCERTAINTY_MEASURE_WITH_UNIT(LENGTH_MEASURE(0.001),#85790,
'DISTANCE_ACCURACY_VALUE',
'Maximum model space distance between geometric entities at asserted c
onnectivities');
#85769=UNCERTAINTY_MEASURE_WITH_UNIT(LENGTH_MEASURE(0.001),#85790,
'DISTANCE_ACCURACY_VALUE',
'Maximum model space distance between geometric entities at asserted c
onnectivities');
#85787=(
GEOMETRIC_REPRESENTATION_CONTEXT(3)
GLOBAL_UNCERTAINTY_ASSIGNED_CONTEXT((#85767))
GLOBAL_UNIT_ASSIGNED_CONTEXT((#85790,#85792,#85793))
REPRESENTATION_CONTEXT('','3D')
);
#85789=(
GEOMETRIC_REPRESENTATION_CONTEXT(3)
GLOBAL_UNCERTAINTY_ASSIGNED_CONTEXT((#85769))
GLOBAL_UNIT_ASSIGNED_CONTEXT((#85790,#85792,#85793))
REPRESENTATION_CONTEXT('','3D')
);
#85790=(
LENGTH_UNIT()
NAMED_UNIT(*)
SI_UNIT(.CENTI.,.METRE.)
);
#85792=(
NAMED_UNIT(*)
PLANE_ANGLE_UNIT()
SI_UNIT($,.RADIAN.)
);
#85793=(
NAMED_UNIT(*)
SI_UNIT($,.STERADIAN.)
SOLID_ANGLE_UNIT()
);
#85811=SHAPE_DEFINITION_REPRESENTATION(#85830,#85879);
#85830=PRODUCT_DEFINITION_SHAPE('',$,#85899);
#85879=SHAPE_REPRESENTATION('',(#10855),#85787);
#85881=PRODUCT_DEFINITION_CONTEXT('part definition',#85940,'design');
#85899=PRODUCT_DEFINITION('DIN 6799 E-Ring 5','DIN 6799 E-Ring 5',#85918,
#85881);
#85918=PRODUCT_DEFINITION_FORMATION('',$,#85959);
#85940=APPLICATION_CONTEXT(
'Core Data for Automotive Mechanical Design Process');
#85941=PRODUCT_CONTEXT('part definition',#85940,'mechanical');
#85959=PRODUCT('DIN 6799 E-Ring 5','DIN 6799 E-Ring 5',$,(#85941));
#85978=PRESENTATION_STYLE_ASSIGNMENT((#85996));
#85996=SURFACE_STYLE_USAGE(.BOTH.,#86014);
#86014=SURFACE_SIDE_STYLE('',(#86032));
#86032=SURFACE_STYLE_FILL_AREA(#86050);
#86050=FILL_AREA_STYLE('Opaque(198,202,207)',(#86068));
#86068=FILL_AREA_STYLE_COLOUR('Opaque(198,202,207)',#86086);
#86086=COLOUR_RGB('Opaque(198,202,207)', 0.08235294, 0.09019608, 0.10196078);
ENDSEC;
END-ISO-10303-21;
